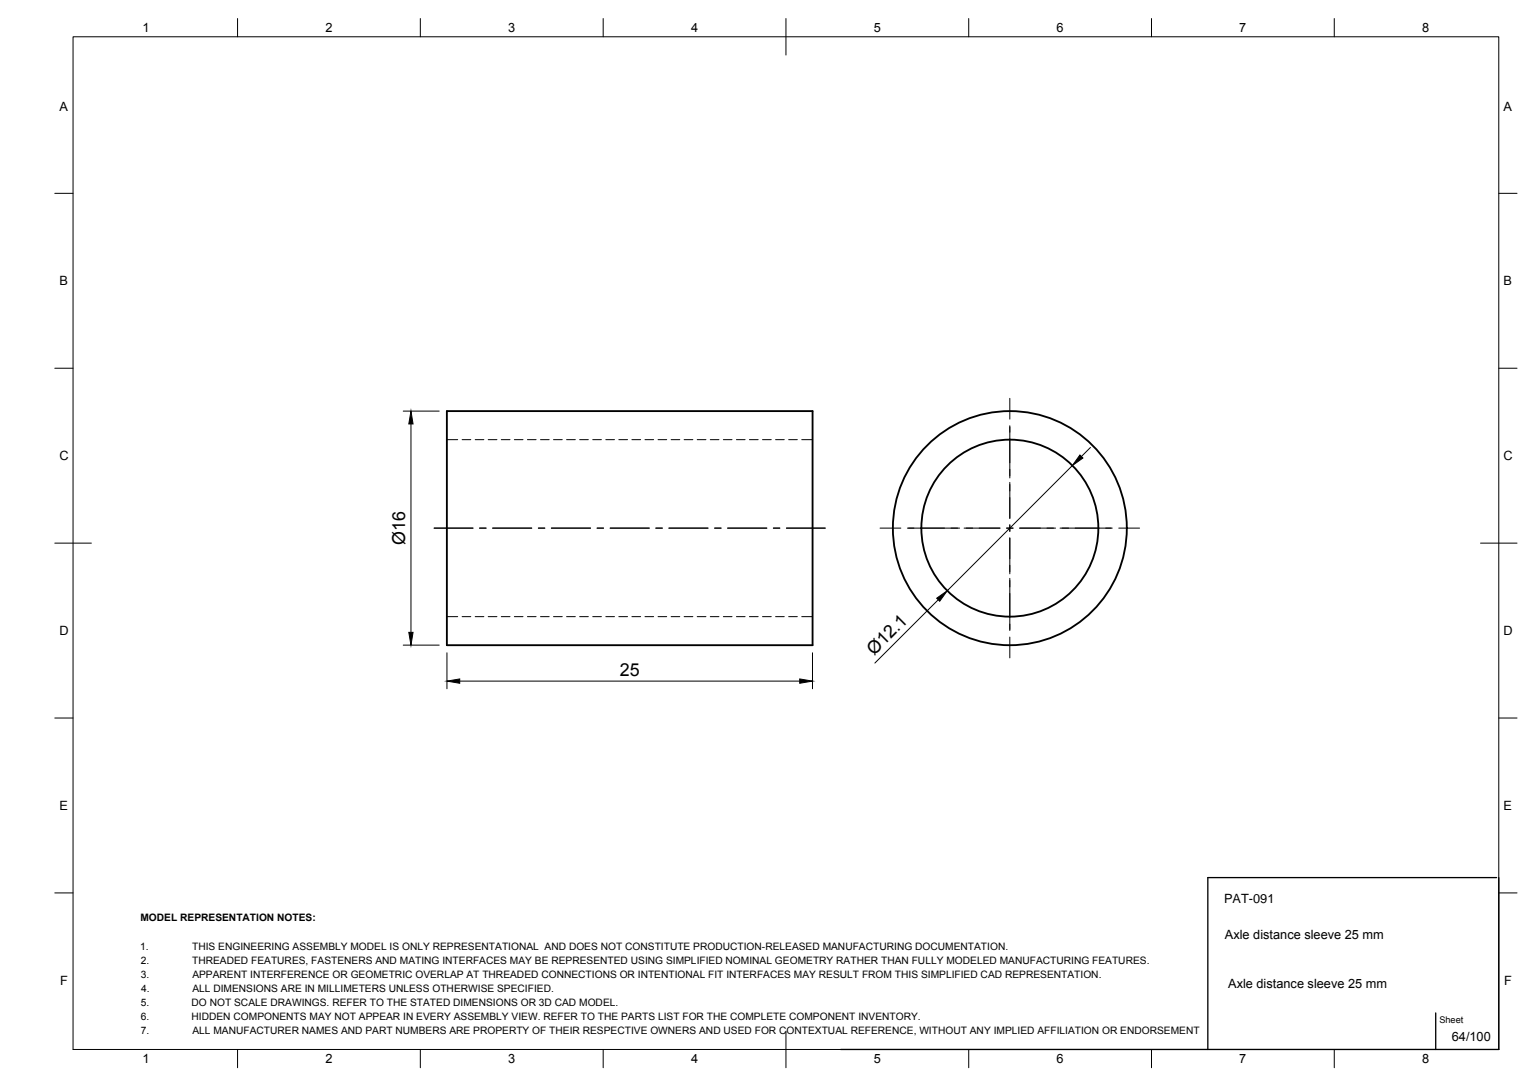
ISO-10303-21;
HEADER;
/* Generated by software containing ST-Developer
 * from STEP Tools, Inc. (www.steptools.com) 
 */

FILE_DESCRIPTION(
/* description */ ('PAT-091'),
/* implementation_level */ '2;1');

FILE_NAME(
/* name */ 'Axle distance sleeve 25 mm.step',
/* time_stamp */ '2026-10-27T15:34:44-07:00',
/* author */ (''),
/* organization */ (''),
/* preprocessor_version */ 'ST-DEVELOPER v20.2',
/* originating_system */ 'Autodesk Translation Framework v15.17.0.0',
/* authorisation */ '');

FILE_SCHEMA (('AUTOMOTIVE_DESIGN { 1 0 10303 214 3 1 1 }'));
ENDSEC;

DATA;
#10=MECHANICAL_DESIGN_GEOMETRIC_PRESENTATION_REPRESENTATION('',(#1021),#25100);
#801=SHAPE_REPRESENTATION_RELATIONSHIP('SRR','None',#25565,#911);
#911=ADVANCED_BREP_SHAPE_REPRESENTATION('',(#1143),#25035);
#1021=STYLED_ITEM('',(#26191),#1143);
#1143=MANIFOLD_SOLID_BREP('Body1',#13300);
#1466=FACE_BOUND('',#3535,.T.);
#1467=FACE_BOUND('',#3537,.T.);
#1863=PLANE('',#15398);
#1864=PLANE('',#15399);
#2463=FACE_OUTER_BOUND('',#3532,.T.);
#2464=FACE_OUTER_BOUND('',#3533,.T.);
#2465=FACE_OUTER_BOUND('',#3534,.T.);
#2466=FACE_OUTER_BOUND('',#3536,.T.);
#3532=EDGE_LOOP('',(#10596,#10597,#10598,#10599));
#3533=EDGE_LOOP('',(#10600,#10601,#10602,#10603));
#3534=EDGE_LOOP('',(#10604));
#3535=EDGE_LOOP('',(#10605));
#3536=EDGE_LOOP('',(#10606));
#3537=EDGE_LOOP('',(#10607));
#4581=LINE('',#22837,#5321);
#4582=LINE('',#22843,#5322);
#5321=VECTOR('',#18543,0.604999999999997);
#5322=VECTOR('',#18550,0.799999999999997);
#5955=CIRCLE('',#15393,0.604999999999997);
#5956=CIRCLE('',#15394,0.604999999999997);
#5957=CIRCLE('',#15396,0.799999999999997);
#5958=CIRCLE('',#15397,0.799999999999997);
#6922=VERTEX_POINT('',#22834);
#6923=VERTEX_POINT('',#22836);
#6924=VERTEX_POINT('',#22840);
#6925=VERTEX_POINT('',#22842);
#8233=EDGE_CURVE('',#6922,#6922,#5955,.T.);
#8234=EDGE_CURVE('',#6922,#6923,#4581,.T.);
#8235=EDGE_CURVE('',#6923,#6923,#5956,.T.);
#8236=EDGE_CURVE('',#6924,#6924,#5957,.T.);
#8237=EDGE_CURVE('',#6924,#6925,#4582,.T.);
#8238=EDGE_CURVE('',#6925,#6925,#5958,.T.);
#10596=ORIENTED_EDGE('',*,*,#8233,.F.);
#10597=ORIENTED_EDGE('',*,*,#8234,.T.);
#10598=ORIENTED_EDGE('',*,*,#8235,.T.);
#10599=ORIENTED_EDGE('',*,*,#8234,.F.);
#10600=ORIENTED_EDGE('',*,*,#8236,.F.);
#10601=ORIENTED_EDGE('',*,*,#8237,.T.);
#10602=ORIENTED_EDGE('',*,*,#8238,.T.);
#10603=ORIENTED_EDGE('',*,*,#8237,.F.);
#10604=ORIENTED_EDGE('',*,*,#8236,.T.);
#10605=ORIENTED_EDGE('',*,*,#8233,.T.);
#10606=ORIENTED_EDGE('',*,*,#8238,.F.);
#10607=ORIENTED_EDGE('',*,*,#8235,.F.);
#12244=CYLINDRICAL_SURFACE('',#15392,0.604999999999997);
#12245=CYLINDRICAL_SURFACE('',#15395,0.799999999999997);
#12830=ADVANCED_FACE('',(#2463),#12244,.F.);
#12831=ADVANCED_FACE('',(#2464),#12245,.T.);
#12832=ADVANCED_FACE('',(#2465,#1466),#1863,.T.);
#12833=ADVANCED_FACE('',(#2466,#1467),#1864,.F.);
#13300=CLOSED_SHELL('',(#12830,#12831,#12832,#12833));
#15391=AXIS2_PLACEMENT_3D('',#22832,#18537,#18538);
#15392=AXIS2_PLACEMENT_3D('',#22833,#18539,#18540);
#15393=AXIS2_PLACEMENT_3D('',#22835,#18541,#18542);
#15394=AXIS2_PLACEMENT_3D('',#22838,#18544,#18545);
#15395=AXIS2_PLACEMENT_3D('',#22839,#18546,#18547);
#15396=AXIS2_PLACEMENT_3D('',#22841,#18548,#18549);
#15397=AXIS2_PLACEMENT_3D('',#22844,#18551,#18552);
#15398=AXIS2_PLACEMENT_3D('',#22845,#18553,#18554);
#15399=AXIS2_PLACEMENT_3D('',#22846,#18555,#18556);
#18537=DIRECTION('axis',(0.,0.,1.));
#18538=DIRECTION('refdir',(1.,0.,0.));
#18539=DIRECTION('center_axis',(0.,1.,0.));
#18540=DIRECTION('ref_axis',(1.,0.,0.));
#18541=DIRECTION('center_axis',(0.,-1.,0.));
#18542=DIRECTION('ref_axis',(1.,0.,0.));
#18543=DIRECTION('',(0.,-1.,0.));
#18544=DIRECTION('center_axis',(0.,-1.,0.));
#18545=DIRECTION('ref_axis',(1.,0.,0.));
#18546=DIRECTION('center_axis',(0.,1.,0.));
#18547=DIRECTION('ref_axis',(1.,0.,0.));
#18548=DIRECTION('center_axis',(0.,1.,0.));
#18549=DIRECTION('ref_axis',(1.,0.,0.));
#18550=DIRECTION('',(0.,-1.,0.));
#18551=DIRECTION('center_axis',(0.,1.,0.));
#18552=DIRECTION('ref_axis',(1.,0.,0.));
#18553=DIRECTION('center_axis',(0.,1.,0.));
#18554=DIRECTION('ref_axis',(1.,0.,0.));
#18555=DIRECTION('center_axis',(0.,1.,0.));
#18556=DIRECTION('ref_axis',(1.,0.,0.));
#22832=CARTESIAN_POINT('',(0.,0.,0.));
#22833=CARTESIAN_POINT('Origin',(38.7298334620742,-6.,13.));
#22834=CARTESIAN_POINT('',(38.1248334620742,-3.5,13.));
#22835=CARTESIAN_POINT('Origin',(38.7298334620742,-3.5,13.));
#22836=CARTESIAN_POINT('',(38.1248334620742,-6.,13.));
#22837=CARTESIAN_POINT('',(38.1248334620742,-6.,13.));
#22838=CARTESIAN_POINT('Origin',(38.7298334620742,-6.,13.));
#22839=CARTESIAN_POINT('Origin',(38.7298334620742,-6.,13.));
#22840=CARTESIAN_POINT('',(37.9298334620742,-3.5,13.));
#22841=CARTESIAN_POINT('Origin',(38.7298334620742,-3.5,13.));
#22842=CARTESIAN_POINT('',(37.9298334620742,-6.,13.));
#22843=CARTESIAN_POINT('',(37.9298334620742,-6.,13.));
#22844=CARTESIAN_POINT('Origin',(38.7298334620742,-6.,13.));
#22845=CARTESIAN_POINT('Origin',(38.7298334620742,-3.5,13.));
#22846=CARTESIAN_POINT('Origin',(38.7298334620742,-6.,13.));
#24914=UNCERTAINTY_MEASURE_WITH_UNIT(LENGTH_MEASURE(0.001),#25101,
'DISTANCE_ACCURACY_VALUE',
'Maximum model space distance between geometric entities at asserted c
onnectivities');
#24979=UNCERTAINTY_MEASURE_WITH_UNIT(LENGTH_MEASURE(0.001),#25101,
'DISTANCE_ACCURACY_VALUE',
'Maximum model space distance between geometric entities at asserted c
onnectivities');
#25035=(
GEOMETRIC_REPRESENTATION_CONTEXT(3)
GLOBAL_UNCERTAINTY_ASSIGNED_CONTEXT((#24914))
GLOBAL_UNIT_ASSIGNED_CONTEXT((#25101,#25103,#25104))
REPRESENTATION_CONTEXT('','3D')
);
#25100=(
GEOMETRIC_REPRESENTATION_CONTEXT(3)
GLOBAL_UNCERTAINTY_ASSIGNED_CONTEXT((#24979))
GLOBAL_UNIT_ASSIGNED_CONTEXT((#25101,#25103,#25104))
REPRESENTATION_CONTEXT('','3D')
);
#25101=(
LENGTH_UNIT()
NAMED_UNIT(*)
SI_UNIT(.CENTI.,.METRE.)
);
#25103=(
NAMED_UNIT(*)
PLANE_ANGLE_UNIT()
SI_UNIT($,.RADIAN.)
);
#25104=(
NAMED_UNIT(*)
SI_UNIT($,.STERADIAN.)
SOLID_ANGLE_UNIT()
);
#25160=SHAPE_DEFINITION_REPRESENTATION(#25280,#25565);
#25280=PRODUCT_DEFINITION_SHAPE('',$,#25686);
#25565=SHAPE_REPRESENTATION('',(#15391),#25035);
#25630=PRODUCT_DEFINITION_CONTEXT('part definition',#25992,'design');
#25686=PRODUCT_DEFINITION('Axle distance sleeve 25 mm',
'Axle distance sleeve 25 mm',#25806,#25630);
#25806=PRODUCT_DEFINITION_FORMATION('',$,#26049);
#25992=APPLICATION_CONTEXT(
'Core Data for Automotive Mechanical Design Process');
#25993=PRODUCT_CONTEXT('part definition',#25992,'mechanical');
#26049=PRODUCT('Axle distance sleeve 25 mm',
'Axle distance sleeve 25 mm','Axle distance sleeve 25 mm',(#25993));
#26185=COLOUR_RGB('Grey',0.48,0.52,0.57);
#26186=FILL_AREA_STYLE_COLOUR('',#26185);
#26187=FILL_AREA_STYLE('',(#26186));
#26188=SURFACE_STYLE_FILL_AREA(#26187);
#26189=SURFACE_SIDE_STYLE('',(#26188));
#26190=SURFACE_STYLE_USAGE(.BOTH.,#26189);
#26191=PRESENTATION_STYLE_ASSIGNMENT((#26190));
ENDSEC;
END-ISO-10303-21;
